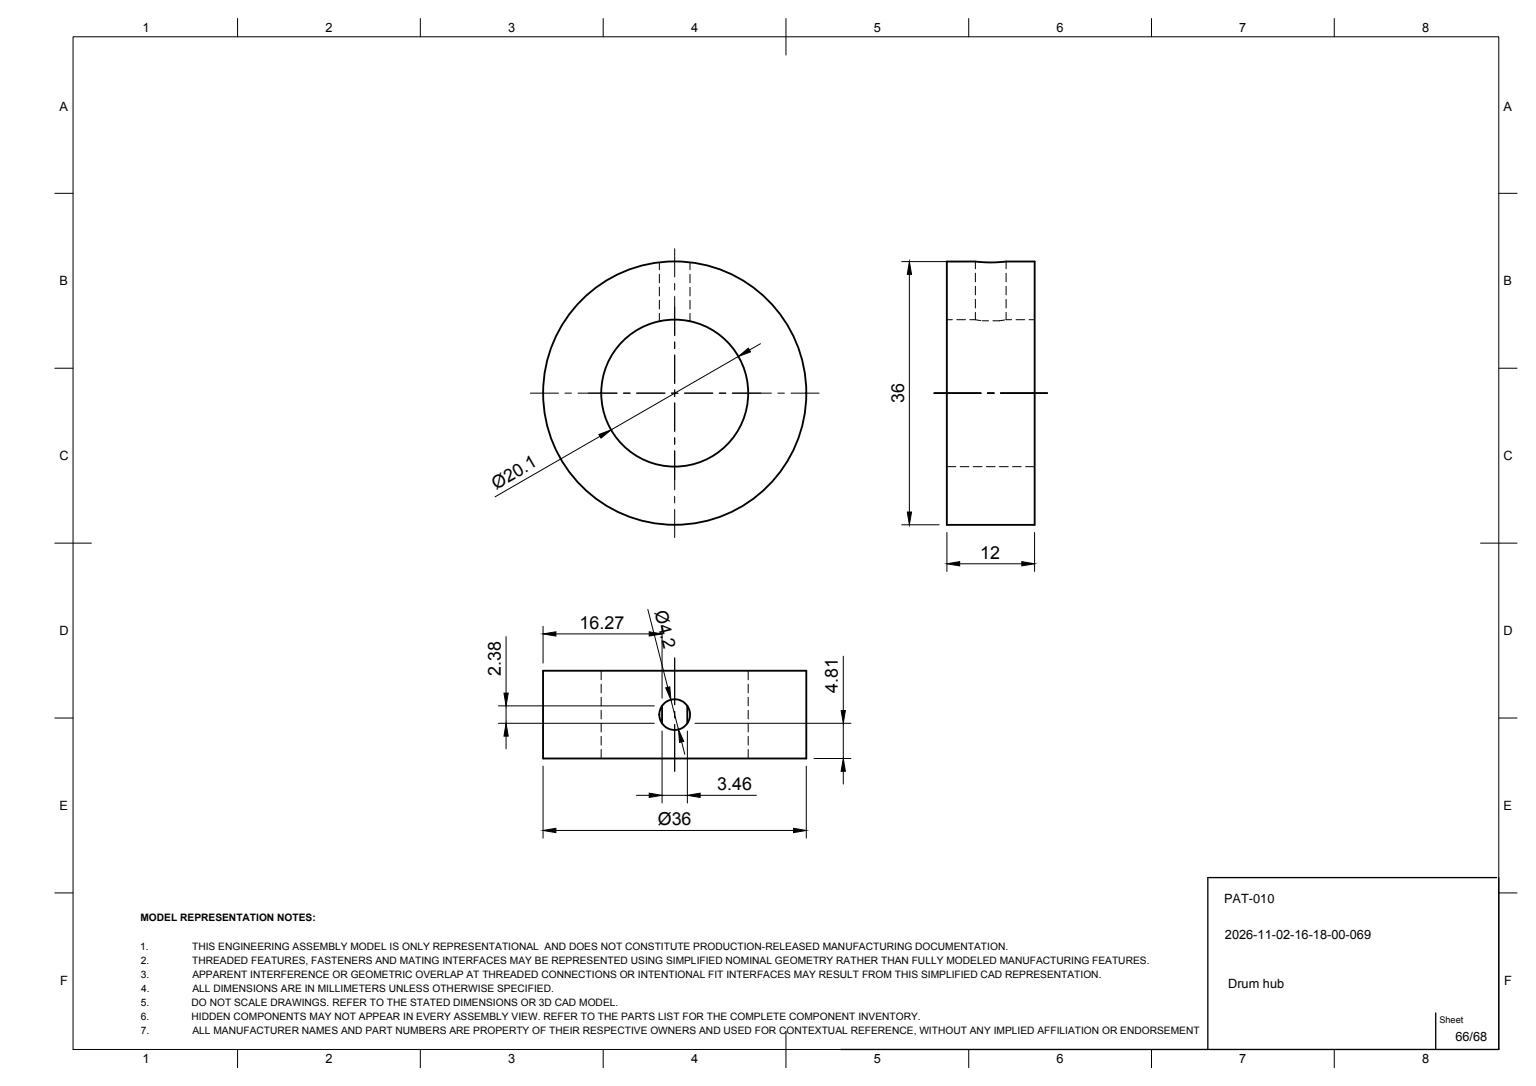
ISO-10303-21;
HEADER;
/* Generated by software containing ST-Developer
 * from STEP Tools, Inc. (www.steptools.com) 
 */

FILE_DESCRIPTION(
/* description */ ('Belt conveyor head drive unit'),
/* implementation_level */ '2;1');

FILE_NAME(
/* name */ 'Drum hub.step',
/* time_stamp */ '2026-10-28T03:26:19-07:00',
/* author */ (''),
/* organization */ (''),
/* preprocessor_version */ 'ST-DEVELOPER v20.2',
/* originating_system */ 'Autodesk Translation Framework v15.17.0.0',
/* authorisation */ '');

FILE_SCHEMA (('AUTOMOTIVE_DESIGN { 1 0 10303 214 3 1 1 }'));
ENDSEC;

DATA;
#10=MECHANICAL_DESIGN_GEOMETRIC_PRESENTATION_REPRESENTATION('',(#927),#27069);
#615=B_SPLINE_CURVE_WITH_KNOTS('',3,(#25655,#25656,#25657,#25658,#25659,
#25660,#25661,#25662,#25663,#25664,#25665,#25666,#25667,#25668),
 .UNSPECIFIED.,.F.,.F.,(4,2,2,2,2,2,4),(0.756005737987022,0.793568827564647,
0.872922520054202,0.952276212543756,1.03162990503331,1.11098359752287,1.14854668710049),
 .UNSPECIFIED.);
#616=B_SPLINE_CURVE_WITH_KNOTS('',3,(#25674,#25675,#25676,#25677,#25678,
#25679,#25680,#25681,#25682,#25683,#25684,#25685,#25686,#25687,#25688,#25689,
#25690,#25691),.UNSPECIFIED.,.F.,.F.,(4,2,2,2,2,2,2,2,4),(0.,0.079181905547237,
0.158363811094474,0.237545215630596,0.316726620166717,0.395908024702839,
0.47508942923896,0.554271334786198,0.633453240333435),.UNSPECIFIED.);
#617=B_SPLINE_CURVE_WITH_KNOTS('',3,(#25692,#25693,#25694,#25695,#25696,
#25697,#25698,#25699,#25700,#25701,#25702,#25703,#25704,#25705,#25706,#25707,
#25708,#25709),.UNSPECIFIED.,.F.,.F.,(4,2,2,2,2,2,2,2,4),(0.633453240333435,
0.712635145880671,0.791817051427908,0.87099845596403,0.950179860500152,
1.02936126503627,1.1085426695724,1.18772457511963,1.26690648066687),
 .UNSPECIFIED.);
#618=B_SPLINE_CURVE_WITH_KNOTS('',3,(#25712,#25713,#25714,#25715,#25716,
#25717,#25718,#25719,#25720,#25721,#25722,#25723,#25724,#25725),
 .UNSPECIFIED.,.F.,.F.,(4,2,2,2,2,2,4),(0.121154929624519,0.158718019202143,
0.238071711691698,0.317425404181252,0.396779096670806,0.476132789160361,
0.513695878737986),.UNSPECIFIED.);
#773=SHAPE_REPRESENTATION_RELATIONSHIP('SRR','None',#27422,#842);
#842=ADVANCED_BREP_SHAPE_REPRESENTATION('',(#1008),#27064);
#927=STYLED_ITEM('',(#27783),#1008);
#1008=MANIFOLD_SOLID_BREP('Body1',#13796);
#1256=FACE_BOUND('',#3345,.T.);
#1257=FACE_BOUND('',#3347,.T.);
#1258=FACE_BOUND('',#3349,.T.);
#1259=FACE_BOUND('',#3351,.T.);
#1600=PLANE('',#15987);
#1601=PLANE('',#15992);
#1602=PLANE('',#15999);
#1603=PLANE('',#16000);
#2297=FACE_OUTER_BOUND('',#3341,.T.);
#2298=FACE_OUTER_BOUND('',#3342,.T.);
#2299=FACE_OUTER_BOUND('',#3343,.T.);
#2300=FACE_OUTER_BOUND('',#3344,.T.);
#2301=FACE_OUTER_BOUND('',#3346,.T.);
#2302=FACE_OUTER_BOUND('',#3348,.T.);
#2303=FACE_OUTER_BOUND('',#3350,.T.);
#3341=EDGE_LOOP('',(#11794,#11795));
#3342=EDGE_LOOP('',(#11796,#11797,#11798,#11799,#11800,#11801,#11802,#11803,
#11804));
#3343=EDGE_LOOP('',(#11805,#11806,#11807));
#3344=EDGE_LOOP('',(#11808,#11809,#11810,#11811));
#3345=EDGE_LOOP('',(#11812,#11813,#11814,#11815));
#3346=EDGE_LOOP('',(#11816,#11817,#11818,#11819));
#3347=EDGE_LOOP('',(#11820,#11821));
#3348=EDGE_LOOP('',(#11822));
#3349=EDGE_LOOP('',(#11823));
#3350=EDGE_LOOP('',(#11824));
#3351=EDGE_LOOP('',(#11825));
#4145=LINE('',#25651,#4937);
#4146=LINE('',#25672,#4938);
#4147=LINE('',#25727,#4939);
#4148=LINE('',#25732,#4940);
#4149=LINE('',#25738,#4941);
#4937=VECTOR('',#19933,1.);
#4938=VECTOR('',#19940,0.21);
#4939=VECTOR('',#19945,1.);
#4940=VECTOR('',#19950,1.005);
#4941=VECTOR('',#19957,1.8);
#5759=CIRCLE('',#15988,0.21);
#5760=CIRCLE('',#15990,0.21);
#5761=CIRCLE('',#15991,0.21);
#5762=CIRCLE('',#15994,1.005);
#5763=CIRCLE('',#15995,1.005);
#5764=CIRCLE('',#15997,1.8);
#5765=CIRCLE('',#15998,1.8);
#6923=VERTEX_POINT('',#25649);
#6924=VERTEX_POINT('',#25650);
#6925=VERTEX_POINT('',#25654);
#6926=VERTEX_POINT('',#25669);
#6927=VERTEX_POINT('',#25671);
#6928=VERTEX_POINT('',#25673);
#6929=VERTEX_POINT('',#25710);
#6930=VERTEX_POINT('',#25729);
#6931=VERTEX_POINT('',#25731);
#6932=VERTEX_POINT('',#25735);
#6933=VERTEX_POINT('',#25737);
#8589=EDGE_CURVE('',#6923,#6924,#4145,.T.);
#8590=EDGE_CURVE('',#6923,#6924,#5759,.T.);
#8591=EDGE_CURVE('',#6925,#6923,#615,.T.);
#8592=EDGE_CURVE('',#6926,#6925,#5760,.T.);
#8593=EDGE_CURVE('',#6926,#6927,#4146,.T.);
#8594=EDGE_CURVE('',#6928,#6927,#616,.T.);
#8595=EDGE_CURVE('',#6927,#6928,#617,.T.);
#8596=EDGE_CURVE('',#6929,#6926,#5761,.T.);
#8597=EDGE_CURVE('',#6924,#6929,#618,.T.);
#8598=EDGE_CURVE('',#6929,#6925,#4147,.T.);
#8599=EDGE_CURVE('',#6930,#6930,#5762,.T.);
#8600=EDGE_CURVE('',#6930,#6931,#4148,.T.);
#8601=EDGE_CURVE('',#6931,#6931,#5763,.T.);
#8602=EDGE_CURVE('',#6932,#6932,#5764,.T.);
#8603=EDGE_CURVE('',#6932,#6933,#4149,.T.);
#8604=EDGE_CURVE('',#6933,#6933,#5765,.T.);
#11794=ORIENTED_EDGE('',*,*,#8589,.F.);
#11795=ORIENTED_EDGE('',*,*,#8590,.T.);
#11796=ORIENTED_EDGE('',*,*,#8591,.F.);
#11797=ORIENTED_EDGE('',*,*,#8592,.F.);
#11798=ORIENTED_EDGE('',*,*,#8593,.T.);
#11799=ORIENTED_EDGE('',*,*,#8594,.F.);
#11800=ORIENTED_EDGE('',*,*,#8595,.F.);
#11801=ORIENTED_EDGE('',*,*,#8593,.F.);
#11802=ORIENTED_EDGE('',*,*,#8596,.F.);
#11803=ORIENTED_EDGE('',*,*,#8597,.F.);
#11804=ORIENTED_EDGE('',*,*,#8590,.F.);
#11805=ORIENTED_EDGE('',*,*,#8598,.F.);
#11806=ORIENTED_EDGE('',*,*,#8596,.T.);
#11807=ORIENTED_EDGE('',*,*,#8592,.T.);
#11808=ORIENTED_EDGE('',*,*,#8599,.F.);
#11809=ORIENTED_EDGE('',*,*,#8600,.T.);
#11810=ORIENTED_EDGE('',*,*,#8601,.T.);
#11811=ORIENTED_EDGE('',*,*,#8600,.F.);
#11812=ORIENTED_EDGE('',*,*,#8597,.T.);
#11813=ORIENTED_EDGE('',*,*,#8598,.T.);
#11814=ORIENTED_EDGE('',*,*,#8591,.T.);
#11815=ORIENTED_EDGE('',*,*,#8589,.T.);
#11816=ORIENTED_EDGE('',*,*,#8602,.F.);
#11817=ORIENTED_EDGE('',*,*,#8603,.T.);
#11818=ORIENTED_EDGE('',*,*,#8604,.T.);
#11819=ORIENTED_EDGE('',*,*,#8603,.F.);
#11820=ORIENTED_EDGE('',*,*,#8594,.T.);
#11821=ORIENTED_EDGE('',*,*,#8595,.T.);
#11822=ORIENTED_EDGE('',*,*,#8602,.T.);
#11823=ORIENTED_EDGE('',*,*,#8599,.T.);
#11824=ORIENTED_EDGE('',*,*,#8604,.F.);
#11825=ORIENTED_EDGE('',*,*,#8601,.F.);
#12815=CYLINDRICAL_SURFACE('',#15989,0.21);
#12816=CYLINDRICAL_SURFACE('',#15993,1.005);
#12817=CYLINDRICAL_SURFACE('',#15996,1.8);
#13576=ADVANCED_FACE('',(#2297),#1600,.T.);
#13577=ADVANCED_FACE('',(#2298),#12815,.F.);
#13578=ADVANCED_FACE('',(#2299),#1601,.T.);
#13579=ADVANCED_FACE('',(#2300,#1256),#12816,.F.);
#13580=ADVANCED_FACE('',(#2301,#1257),#12817,.T.);
#13581=ADVANCED_FACE('',(#2302,#1258),#1602,.T.);
#13582=ADVANCED_FACE('',(#2303,#1259),#1603,.F.);
#13796=CLOSED_SHELL('',(#13576,#13577,#13578,#13579,#13580,#13581,#13582));
#15986=AXIS2_PLACEMENT_3D('',#25647,#19929,#19930);
#15987=AXIS2_PLACEMENT_3D('',#25648,#19931,#19932);
#15988=AXIS2_PLACEMENT_3D('',#25652,#19934,#19935);
#15989=AXIS2_PLACEMENT_3D('',#25653,#19936,#19937);
#15990=AXIS2_PLACEMENT_3D('',#25670,#19938,#19939);
#15991=AXIS2_PLACEMENT_3D('',#25711,#19941,#19942);
#15992=AXIS2_PLACEMENT_3D('',#25726,#19943,#19944);
#15993=AXIS2_PLACEMENT_3D('',#25728,#19946,#19947);
#15994=AXIS2_PLACEMENT_3D('',#25730,#19948,#19949);
#15995=AXIS2_PLACEMENT_3D('',#25733,#19951,#19952);
#15996=AXIS2_PLACEMENT_3D('',#25734,#19953,#19954);
#15997=AXIS2_PLACEMENT_3D('',#25736,#19955,#19956);
#15998=AXIS2_PLACEMENT_3D('',#25739,#19958,#19959);
#15999=AXIS2_PLACEMENT_3D('',#25740,#19960,#19961);
#16000=AXIS2_PLACEMENT_3D('',#25741,#19962,#19963);
#19929=DIRECTION('axis',(0.,0.,1.));
#19930=DIRECTION('refdir',(1.,0.,0.));
#19931=DIRECTION('center_axis',(0.,0.,1.));
#19932=DIRECTION('ref_axis',(1.,0.,0.));
#19933=DIRECTION('',(0.,1.,0.));
#19934=DIRECTION('center_axis',(0.,0.,1.));
#19935=DIRECTION('ref_axis',(1.,0.,0.));
#19936=DIRECTION('center_axis',(0.,0.,1.));
#19937=DIRECTION('ref_axis',(1.,0.,0.));
#19938=DIRECTION('center_axis',(0.,0.,1.));
#19939=DIRECTION('ref_axis',(1.,0.,0.));
#19940=DIRECTION('',(0.,0.,1.));
#19941=DIRECTION('center_axis',(0.,0.,1.));
#19942=DIRECTION('ref_axis',(1.,0.,0.));
#19943=DIRECTION('center_axis',(0.,0.,1.));
#19944=DIRECTION('ref_axis',(1.,0.,0.));
#19945=DIRECTION('',(0.,-1.,0.));
#19946=DIRECTION('center_axis',(0.,1.,0.));
#19947=DIRECTION('ref_axis',(1.,0.,0.));
#19948=DIRECTION('center_axis',(0.,-1.,0.));
#19949=DIRECTION('ref_axis',(1.,0.,0.));
#19950=DIRECTION('',(0.,-1.,0.));
#19951=DIRECTION('center_axis',(0.,-1.,0.));
#19952=DIRECTION('ref_axis',(1.,0.,0.));
#19953=DIRECTION('center_axis',(0.,1.,0.));
#19954=DIRECTION('ref_axis',(1.,0.,0.));
#19955=DIRECTION('center_axis',(0.,1.,0.));
#19956=DIRECTION('ref_axis',(1.,0.,0.));
#19957=DIRECTION('',(0.,-1.,0.));
#19958=DIRECTION('center_axis',(0.,1.,0.));
#19959=DIRECTION('ref_axis',(1.,0.,0.));
#19960=DIRECTION('center_axis',(0.,1.,0.));
#19961=DIRECTION('ref_axis',(1.,0.,0.));
#19962=DIRECTION('center_axis',(0.,1.,0.));
#19963=DIRECTION('ref_axis',(1.,0.,0.));
#25647=CARTESIAN_POINT('',(0.,0.,0.));
#25648=CARTESIAN_POINT('Origin',(6.97091003018116,7.6,7.99));
#25649=CARTESIAN_POINT('',(7.14389846910121,7.48094119100208,7.99));
#25650=CARTESIAN_POINT('',(7.14389846910121,7.71905880899792,7.99));
#25651=CARTESIAN_POINT('',(7.14389846910121,7.,7.99));
#25652=CARTESIAN_POINT('Origin',(6.97091003018116,7.6,7.99));
#25653=CARTESIAN_POINT('Origin',(6.97091003018116,7.6,7.99));
#25654=CARTESIAN_POINT('',(6.7979215912611,7.48094119100208,7.99));
#25655=CARTESIAN_POINT('Ctrl Pts',(6.7979215912611,7.48094119100208,7.99));
#25656=CARTESIAN_POINT('Ctrl Pts',(6.80531516486984,7.47019857760471,7.99129192197638));
#25657=CARTESIAN_POINT('Ctrl Pts',(6.81361289145555,7.46031229062725,7.99265394943905));
#25658=CARTESIAN_POINT('Ctrl Pts',(6.84101795633608,7.43290722574673,7.9967480843909));
#25659=CARTESIAN_POINT('Ctrl Pts',(6.86457986242187,7.41675794366705,7.99969589327638));
#25660=CARTESIAN_POINT('Ctrl Pts',(6.91629712554875,7.39530220603509,8.00385029472357));
#25661=CARTESIAN_POINT('Ctrl Pts',(6.9444587993513,7.39,8.005));
#25662=CARTESIAN_POINT('Ctrl Pts',(6.99736126101101,7.39,8.005));
#25663=CARTESIAN_POINT('Ctrl Pts',(7.02552293481356,7.39530220603509,8.00385029472357));
#25664=CARTESIAN_POINT('Ctrl Pts',(7.07724019794044,7.41675794366705,7.99969589327638));
#25665=CARTESIAN_POINT('Ctrl Pts',(7.10080210402623,7.43290722574673,7.9967480843909));
#25666=CARTESIAN_POINT('Ctrl Pts',(7.12820716890676,7.46031229062725,7.99265394943905));
#25667=CARTESIAN_POINT('Ctrl Pts',(7.13650489549247,7.47019857760471,7.99129192197638));
#25668=CARTESIAN_POINT('Ctrl Pts',(7.14389846910121,7.48094119100208,7.99));
#25669=CARTESIAN_POINT('',(6.76091003018116,7.6,7.99));
#25670=CARTESIAN_POINT('Origin',(6.97091003018116,7.6,7.99));
#25671=CARTESIAN_POINT('',(6.76091003018116,7.6,8.78770802985275));
#25672=CARTESIAN_POINT('',(6.76091003018116,7.6,7.99));
#25673=CARTESIAN_POINT('',(7.18091003018116,7.6,8.78770802985275));
#25674=CARTESIAN_POINT('Ctrl Pts',(7.18091003018116,7.6,8.78770802985275));
#25675=CARTESIAN_POINT('Ctrl Pts',(7.18091003018116,7.57360603148425,8.78770802985275));
#25676=CARTESIAN_POINT('Ctrl Pts',(7.17563026313288,7.54546934556601,8.78835284034214));
#25677=CARTESIAN_POINT('Ctrl Pts',(7.15419155416006,7.49373688397397,8.79067700538683));
#25678=CARTESIAN_POINT('Ctrl Pts',(7.13803391906352,7.47013904078401,8.79232226897314));
#25679=CARTESIAN_POINT('Ctrl Pts',(7.10077110728482,7.43287622900531,8.79540680803063));
#25680=CARTESIAN_POINT('Ctrl Pts',(7.07717321270923,7.4167185016358,8.79704717240673));
#25681=CARTESIAN_POINT('Ctrl Pts',(7.02544057769236,7.39527972468261,8.79936011492601));
#25682=CARTESIAN_POINT('Ctrl Pts',(6.9973038316932,7.39,8.8));
#25683=CARTESIAN_POINT('Ctrl Pts',(6.94451622866912,7.39,8.8));
#25684=CARTESIAN_POINT('Ctrl Pts',(6.91637948266995,7.39527972468261,8.79936011492601));
#25685=CARTESIAN_POINT('Ctrl Pts',(6.86464684765309,7.4167185016358,8.79704717240673));
#25686=CARTESIAN_POINT('Ctrl Pts',(6.84104895307749,7.43287622900531,8.79540680803063));
#25687=CARTESIAN_POINT('Ctrl Pts',(6.80378614129879,7.47013904078401,8.79232226897314));
#25688=CARTESIAN_POINT('Ctrl Pts',(6.78762850620226,7.49373688397397,8.79067700538683));
#25689=CARTESIAN_POINT('Ctrl Pts',(6.76618979722943,7.54546934556601,8.78835284034214));
#25690=CARTESIAN_POINT('Ctrl Pts',(6.76091003018116,7.57360603148426,8.78770802985275));
#25691=CARTESIAN_POINT('Ctrl Pts',(6.76091003018116,7.6,8.78770802985275));
#25692=CARTESIAN_POINT('Ctrl Pts',(6.76091003018116,7.6,8.78770802985275));
#25693=CARTESIAN_POINT('Ctrl Pts',(6.76091003018116,7.62639396851575,8.78770802985275));
#25694=CARTESIAN_POINT('Ctrl Pts',(6.76618979722943,7.65453065443399,8.78835284034214));
#25695=CARTESIAN_POINT('Ctrl Pts',(6.78762850620226,7.70626311602603,8.79067700538683));
#25696=CARTESIAN_POINT('Ctrl Pts',(6.80378614129879,7.72986095921599,8.79232226897314));
#25697=CARTESIAN_POINT('Ctrl Pts',(6.84104895307749,7.76712377099468,8.79540680803063));
#25698=CARTESIAN_POINT('Ctrl Pts',(6.86464684765309,7.78328149836419,8.79704717240673));
#25699=CARTESIAN_POINT('Ctrl Pts',(6.91637948266995,7.80472027531739,8.79936011492601));
#25700=CARTESIAN_POINT('Ctrl Pts',(6.94451622866912,7.81,8.8));
#25701=CARTESIAN_POINT('Ctrl Pts',(6.9973038316932,7.81,8.8));
#25702=CARTESIAN_POINT('Ctrl Pts',(7.02544057769236,7.80472027531739,8.79936011492601));
#25703=CARTESIAN_POINT('Ctrl Pts',(7.07717321270923,7.7832814983642,8.79704717240673));
#25704=CARTESIAN_POINT('Ctrl Pts',(7.10077110728482,7.76712377099468,8.79540680803063));
#25705=CARTESIAN_POINT('Ctrl Pts',(7.13803391906352,7.72986095921599,8.79232226897314));
#25706=CARTESIAN_POINT('Ctrl Pts',(7.15419155416005,7.70626311602603,8.79067700538683));
#25707=CARTESIAN_POINT('Ctrl Pts',(7.17563026313288,7.65453065443398,8.78835284034214));
#25708=CARTESIAN_POINT('Ctrl Pts',(7.18091003018116,7.62639396851574,8.78770802985275));
#25709=CARTESIAN_POINT('Ctrl Pts',(7.18091003018116,7.6,8.78770802985275));
#25710=CARTESIAN_POINT('',(6.7979215912611,7.71905880899792,7.99));
#25711=CARTESIAN_POINT('Origin',(6.97091003018116,7.6,7.99));
#25712=CARTESIAN_POINT('Ctrl Pts',(7.14389846910121,7.71905880899792,7.99));
#25713=CARTESIAN_POINT('Ctrl Pts',(7.13650489549247,7.72980142239529,7.99129192197638));
#25714=CARTESIAN_POINT('Ctrl Pts',(7.12820716890676,7.73968770937274,7.99265394943905));
#25715=CARTESIAN_POINT('Ctrl Pts',(7.10080210402623,7.76709277425327,7.9967480843909));
#25716=CARTESIAN_POINT('Ctrl Pts',(7.07724019794044,7.78324205633295,7.99969589327638));
#25717=CARTESIAN_POINT('Ctrl Pts',(7.02552293481356,7.80469779396491,8.00385029472357));
#25718=CARTESIAN_POINT('Ctrl Pts',(6.99736126101101,7.81,8.005));
#25719=CARTESIAN_POINT('Ctrl Pts',(6.9444587993513,7.81,8.005));
#25720=CARTESIAN_POINT('Ctrl Pts',(6.91629712554875,7.80469779396491,8.00385029472357));
#25721=CARTESIAN_POINT('Ctrl Pts',(6.86457986242187,7.78324205633295,7.99969589327638));
#25722=CARTESIAN_POINT('Ctrl Pts',(6.84101795633608,7.76709277425327,7.9967480843909));
#25723=CARTESIAN_POINT('Ctrl Pts',(6.81361289145555,7.73968770937274,7.99265394943905));
#25724=CARTESIAN_POINT('Ctrl Pts',(6.80531516486984,7.72980142239529,7.99129192197638));
#25725=CARTESIAN_POINT('Ctrl Pts',(6.7979215912611,7.71905880899792,7.99));
#25726=CARTESIAN_POINT('Origin',(6.97091003018116,7.6,7.99));
#25727=CARTESIAN_POINT('',(6.7979215912611,7.,7.99));
#25728=CARTESIAN_POINT('Origin',(6.97091003018116,7.,7.));
#25729=CARTESIAN_POINT('',(5.96591003018116,8.2,7.));
#25730=CARTESIAN_POINT('Origin',(6.97091003018116,8.2,7.));
#25731=CARTESIAN_POINT('',(5.96591003018116,7.,7.));
#25732=CARTESIAN_POINT('',(5.96591003018116,7.,7.));
#25733=CARTESIAN_POINT('Origin',(6.97091003018116,7.,7.));
#25734=CARTESIAN_POINT('Origin',(6.97091003018116,7.,7.));
#25735=CARTESIAN_POINT('',(5.17091003018116,8.2,7.));
#25736=CARTESIAN_POINT('Origin',(6.97091003018116,8.2,7.));
#25737=CARTESIAN_POINT('',(5.17091003018116,7.,7.));
#25738=CARTESIAN_POINT('',(5.17091003018116,7.,7.));
#25739=CARTESIAN_POINT('Origin',(6.97091003018116,7.,7.));
#25740=CARTESIAN_POINT('Origin',(6.97091003018116,8.2,7.));
#25741=CARTESIAN_POINT('Origin',(6.97091003018116,7.,7.));
#26987=UNCERTAINTY_MEASURE_WITH_UNIT(LENGTH_MEASURE(0.001),#27070,
'DISTANCE_ACCURACY_VALUE',
'Maximum model space distance between geometric entities at asserted c
onnectivities');
#26992=UNCERTAINTY_MEASURE_WITH_UNIT(LENGTH_MEASURE(0.001),#27070,
'DISTANCE_ACCURACY_VALUE',
'Maximum model space distance between geometric entities at asserted c
onnectivities');
#27064=(
GEOMETRIC_REPRESENTATION_CONTEXT(3)
GLOBAL_UNCERTAINTY_ASSIGNED_CONTEXT((#26987))
GLOBAL_UNIT_ASSIGNED_CONTEXT((#27070,#27072,#27073))
REPRESENTATION_CONTEXT('','3D')
);
#27069=(
GEOMETRIC_REPRESENTATION_CONTEXT(3)
GLOBAL_UNCERTAINTY_ASSIGNED_CONTEXT((#26992))
GLOBAL_UNIT_ASSIGNED_CONTEXT((#27070,#27072,#27073))
REPRESENTATION_CONTEXT('','3D')
);
#27070=(
LENGTH_UNIT()
NAMED_UNIT(*)
SI_UNIT(.CENTI.,.METRE.)
);
#27072=(
NAMED_UNIT(*)
PLANE_ANGLE_UNIT()
SI_UNIT($,.RADIAN.)
);
#27073=(
NAMED_UNIT(*)
SI_UNIT($,.STERADIAN.)
SOLID_ANGLE_UNIT()
);
#27145=SHAPE_DEFINITION_REPRESENTATION(#27233,#27422);
#27233=PRODUCT_DEFINITION_SHAPE('',$,#27499);
#27422=SHAPE_REPRESENTATION('',(#15986),#27064);
#27427=PRODUCT_DEFINITION_CONTEXT('part definition',#27657,'design');
#27499=PRODUCT_DEFINITION('Drum hub','Drum hub',#27575,#27427);
#27575=PRODUCT_DEFINITION_FORMATION('',$,#27730);
#27657=APPLICATION_CONTEXT(
'Core Data for Automotive Mechanical Design Process');
#27658=PRODUCT_CONTEXT('part definition',#27657,'mechanical');
#27730=PRODUCT('Drum hub','Drum hub','Drum hub',(#27658));
#27777=COLOUR_RGB('Light Blue',0.38,0.62,0.78);
#27778=FILL_AREA_STYLE_COLOUR('',#27777);
#27779=FILL_AREA_STYLE('',(#27778));
#27780=SURFACE_STYLE_FILL_AREA(#27779);
#27781=SURFACE_SIDE_STYLE('',(#27780));
#27782=SURFACE_STYLE_USAGE(.BOTH.,#27781);
#27783=PRESENTATION_STYLE_ASSIGNMENT((#27782));
ENDSEC;
END-ISO-10303-21;
